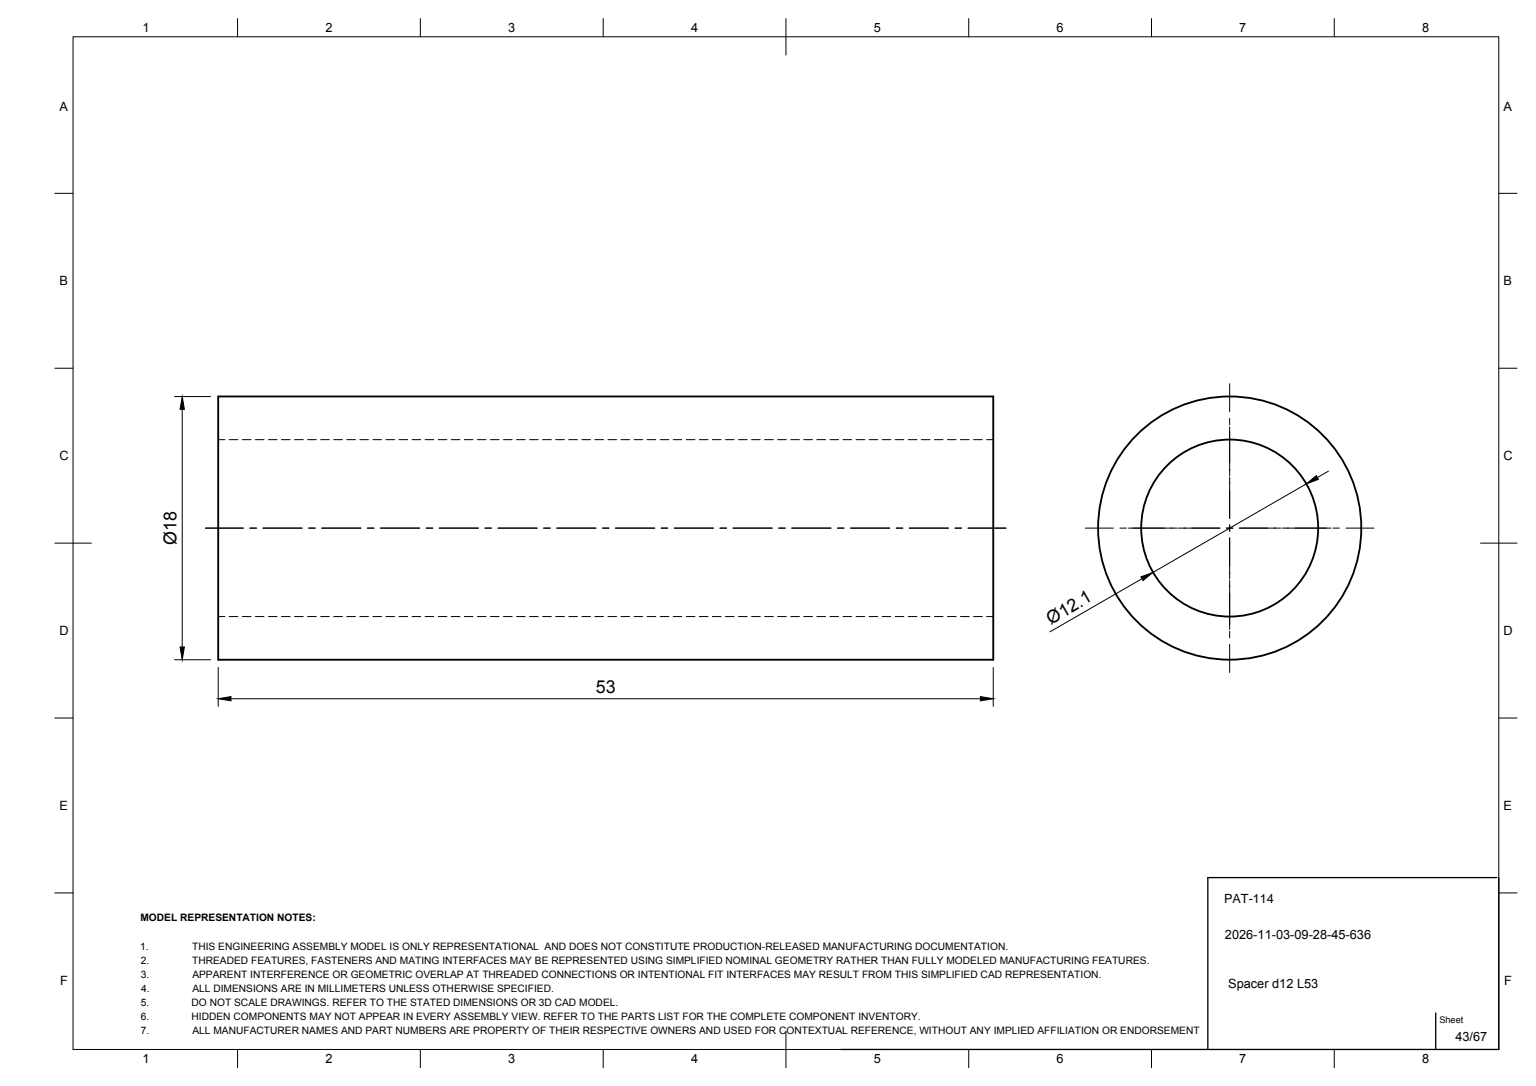
ISO-10303-21;
HEADER;
/* Generated by software containing ST-Developer
 * from STEP Tools, Inc. (www.steptools.com) 
 */

FILE_DESCRIPTION(
/* description */ ('Two-stage gear reducer in split housing'),
/* implementation_level */ '2;1');

FILE_NAME(
/* name */ 'Spacer d12 L53.step',
/* time_stamp */ '2026-10-28T03:22:31-07:00',
/* author */ (''),
/* organization */ (''),
/* preprocessor_version */ 'ST-DEVELOPER v20.2',
/* originating_system */ 'Autodesk Translation Framework v15.17.0.0',
/* authorisation */ '');

FILE_SCHEMA (('AUTOMOTIVE_DESIGN { 1 0 10303 214 3 1 1 }'));
ENDSEC;

DATA;
#10=MECHANICAL_DESIGN_GEOMETRIC_PRESENTATION_REPRESENTATION('',(#1283),#73366);
#1156=SHAPE_REPRESENTATION_RELATIONSHIP('SRR','None',#73646,#1212);
#1212=ADVANCED_BREP_SHAPE_REPRESENTATION('',(#1352),#73342);
#1283=STYLED_ITEM('',(#73981),#1352);
#1352=MANIFOLD_SOLID_BREP('Body1',#16173);
#1553=FACE_BOUND('',#3545,.T.);
#1554=FACE_BOUND('',#3547,.T.);
#1820=PLANE('',#17842);
#1821=PLANE('',#17843);
#2450=FACE_OUTER_BOUND('',#3542,.T.);
#2451=FACE_OUTER_BOUND('',#3543,.T.);
#2452=FACE_OUTER_BOUND('',#3544,.T.);
#2453=FACE_OUTER_BOUND('',#3546,.T.);
#3542=EDGE_LOOP('',(#12419,#12420,#12421,#12422));
#3543=EDGE_LOOP('',(#12423,#12424,#12425,#12426));
#3544=EDGE_LOOP('',(#12427));
#3545=EDGE_LOOP('',(#12428));
#3546=EDGE_LOOP('',(#12429));
#3547=EDGE_LOOP('',(#12430));
#4506=LINE('',#25681,#5530);
#4507=LINE('',#25687,#5531);
#5530=VECTOR('',#20960,0.605);
#5531=VECTOR('',#20967,0.9);
#6570=CIRCLE('',#17837,0.605);
#6571=CIRCLE('',#17838,0.605);
#6572=CIRCLE('',#17840,0.9);
#6573=CIRCLE('',#17841,0.9);
#7477=VERTEX_POINT('',#25678);
#7478=VERTEX_POINT('',#25680);
#7479=VERTEX_POINT('',#25684);
#7480=VERTEX_POINT('',#25686);
#9263=EDGE_CURVE('',#7477,#7477,#6570,.T.);
#9264=EDGE_CURVE('',#7477,#7478,#4506,.T.);
#9265=EDGE_CURVE('',#7478,#7478,#6571,.T.);
#9266=EDGE_CURVE('',#7479,#7479,#6572,.T.);
#9267=EDGE_CURVE('',#7479,#7480,#4507,.T.);
#9268=EDGE_CURVE('',#7480,#7480,#6573,.T.);
#12419=ORIENTED_EDGE('',*,*,#9263,.F.);
#12420=ORIENTED_EDGE('',*,*,#9264,.T.);
#12421=ORIENTED_EDGE('',*,*,#9265,.T.);
#12422=ORIENTED_EDGE('',*,*,#9264,.F.);
#12423=ORIENTED_EDGE('',*,*,#9266,.F.);
#12424=ORIENTED_EDGE('',*,*,#9267,.T.);
#12425=ORIENTED_EDGE('',*,*,#9268,.T.);
#12426=ORIENTED_EDGE('',*,*,#9267,.F.);
#12427=ORIENTED_EDGE('',*,*,#9266,.T.);
#12428=ORIENTED_EDGE('',*,*,#9263,.T.);
#12429=ORIENTED_EDGE('',*,*,#9268,.F.);
#12430=ORIENTED_EDGE('',*,*,#9265,.F.);
#15088=CYLINDRICAL_SURFACE('',#17836,0.605);
#15089=CYLINDRICAL_SURFACE('',#17839,0.9);
#15657=ADVANCED_FACE('',(#2450),#15088,.F.);
#15658=ADVANCED_FACE('',(#2451),#15089,.T.);
#15659=ADVANCED_FACE('',(#2452,#1553),#1820,.T.);
#15660=ADVANCED_FACE('',(#2453,#1554),#1821,.F.);
#16173=CLOSED_SHELL('',(#15657,#15658,#15659,#15660));
#17835=AXIS2_PLACEMENT_3D('',#25676,#20954,#20955);
#17836=AXIS2_PLACEMENT_3D('',#25677,#20956,#20957);
#17837=AXIS2_PLACEMENT_3D('',#25679,#20958,#20959);
#17838=AXIS2_PLACEMENT_3D('',#25682,#20961,#20962);
#17839=AXIS2_PLACEMENT_3D('',#25683,#20963,#20964);
#17840=AXIS2_PLACEMENT_3D('',#25685,#20965,#20966);
#17841=AXIS2_PLACEMENT_3D('',#25688,#20968,#20969);
#17842=AXIS2_PLACEMENT_3D('',#25689,#20970,#20971);
#17843=AXIS2_PLACEMENT_3D('',#25690,#20972,#20973);
#20954=DIRECTION('axis',(0.,0.,1.));
#20955=DIRECTION('refdir',(1.,0.,0.));
#20956=DIRECTION('center_axis',(0.,1.,0.));
#20957=DIRECTION('ref_axis',(1.,0.,0.));
#20958=DIRECTION('center_axis',(0.,-1.,0.));
#20959=DIRECTION('ref_axis',(1.,0.,0.));
#20960=DIRECTION('',(0.,-1.,0.));
#20961=DIRECTION('center_axis',(0.,-1.,0.));
#20962=DIRECTION('ref_axis',(1.,0.,0.));
#20963=DIRECTION('center_axis',(0.,1.,0.));
#20964=DIRECTION('ref_axis',(1.,0.,0.));
#20965=DIRECTION('center_axis',(0.,1.,0.));
#20966=DIRECTION('ref_axis',(1.,0.,0.));
#20967=DIRECTION('',(0.,-1.,0.));
#20968=DIRECTION('center_axis',(0.,1.,0.));
#20969=DIRECTION('ref_axis',(1.,0.,0.));
#20970=DIRECTION('center_axis',(0.,1.,0.));
#20971=DIRECTION('ref_axis',(1.,0.,0.));
#20972=DIRECTION('center_axis',(0.,1.,0.));
#20973=DIRECTION('ref_axis',(1.,0.,0.));
#25676=CARTESIAN_POINT('',(0.,0.,0.));
#25677=CARTESIAN_POINT('Origin',(0.,0.2,10.));
#25678=CARTESIAN_POINT('',(-0.605,5.5,10.));
#25679=CARTESIAN_POINT('Origin',(0.,5.5,10.));
#25680=CARTESIAN_POINT('',(-0.605,0.2,10.));
#25681=CARTESIAN_POINT('',(-0.605,0.2,10.));
#25682=CARTESIAN_POINT('Origin',(0.,0.2,10.));
#25683=CARTESIAN_POINT('Origin',(0.,0.2,10.));
#25684=CARTESIAN_POINT('',(-0.9,5.5,10.));
#25685=CARTESIAN_POINT('Origin',(0.,5.5,10.));
#25686=CARTESIAN_POINT('',(-0.9,0.2,10.));
#25687=CARTESIAN_POINT('',(-0.9,0.2,10.));
#25688=CARTESIAN_POINT('Origin',(0.,0.2,10.));
#25689=CARTESIAN_POINT('Origin',(0.,5.5,10.));
#25690=CARTESIAN_POINT('Origin',(0.,0.2,10.));
#73278=UNCERTAINTY_MEASURE_WITH_UNIT(LENGTH_MEASURE(0.001),#73367,
'DISTANCE_ACCURACY_VALUE',
'Maximum model space distance between geometric entities at asserted c
onnectivities');
#73302=UNCERTAINTY_MEASURE_WITH_UNIT(LENGTH_MEASURE(0.001),#73367,
'DISTANCE_ACCURACY_VALUE',
'Maximum model space distance between geometric entities at asserted c
onnectivities');
#73342=(
GEOMETRIC_REPRESENTATION_CONTEXT(3)
GLOBAL_UNCERTAINTY_ASSIGNED_CONTEXT((#73278))
GLOBAL_UNIT_ASSIGNED_CONTEXT((#73367,#73369,#73370))
REPRESENTATION_CONTEXT('','3D')
);
#73366=(
GEOMETRIC_REPRESENTATION_CONTEXT(3)
GLOBAL_UNCERTAINTY_ASSIGNED_CONTEXT((#73302))
GLOBAL_UNIT_ASSIGNED_CONTEXT((#73367,#73369,#73370))
REPRESENTATION_CONTEXT('','3D')
);
#73367=(
LENGTH_UNIT()
NAMED_UNIT(*)
SI_UNIT(.CENTI.,.METRE.)
);
#73369=(
NAMED_UNIT(*)
PLANE_ANGLE_UNIT()
SI_UNIT($,.RADIAN.)
);
#73370=(
NAMED_UNIT(*)
SI_UNIT($,.STERADIAN.)
SOLID_ANGLE_UNIT()
);
#73410=SHAPE_DEFINITION_REPRESENTATION(#73543,#73646);
#73543=PRODUCT_DEFINITION_SHAPE('',$,#73710);
#73646=SHAPE_REPRESENTATION('',(#17835),#73342);
#73670=PRODUCT_DEFINITION_CONTEXT('part definition',#73861,'design');
#73710=PRODUCT_DEFINITION('Spacer d12 L53','Spacer d12 L53',#73773,#73670);
#73773=PRODUCT_DEFINITION_FORMATION('',$,#73902);
#73861=APPLICATION_CONTEXT(
'Core Data for Automotive Mechanical Design Process');
#73862=PRODUCT_CONTEXT('part definition',#73861,'mechanical');
#73902=PRODUCT('Spacer d12 L53','Spacer d12 L53','Spacer d12 L53',(#73862));
#73975=COLOUR_RGB('Sky Blue',0.24,0.69,0.87);
#73976=FILL_AREA_STYLE_COLOUR('',#73975);
#73977=FILL_AREA_STYLE('',(#73976));
#73978=SURFACE_STYLE_FILL_AREA(#73977);
#73979=SURFACE_SIDE_STYLE('',(#73978));
#73980=SURFACE_STYLE_USAGE(.BOTH.,#73979);
#73981=PRESENTATION_STYLE_ASSIGNMENT((#73980));
ENDSEC;
END-ISO-10303-21;
